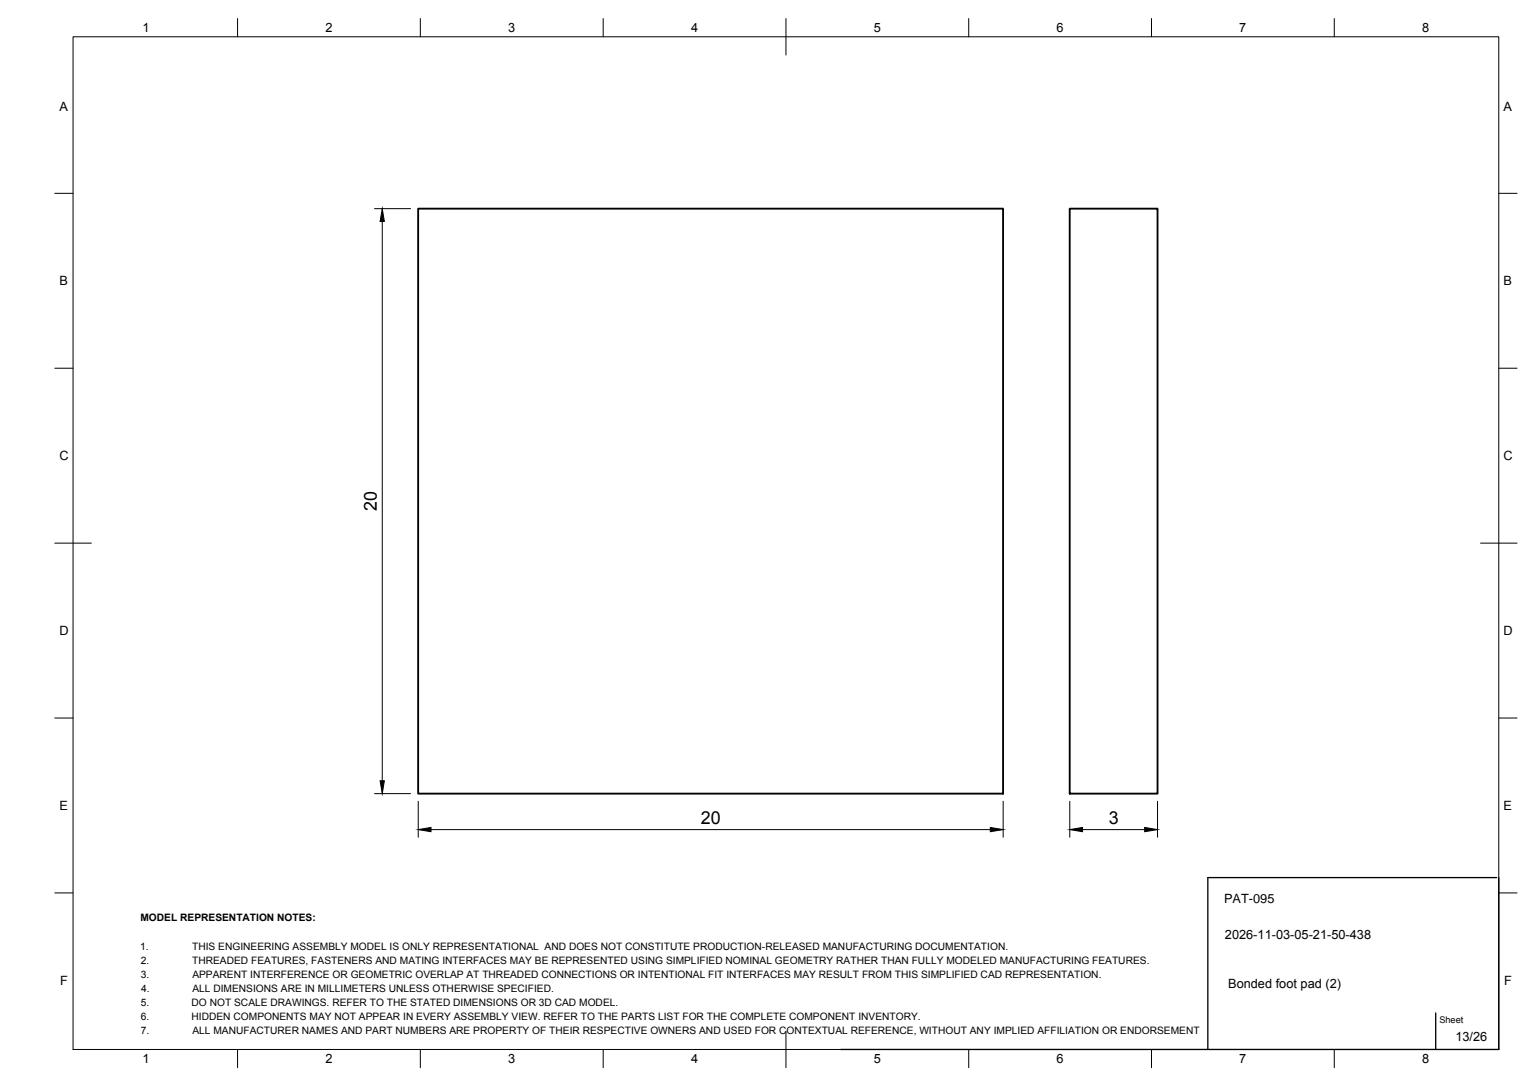
ISO-10303-21;
HEADER;
/* Generated by software containing ST-Developer
 * from STEP Tools, Inc. (www.steptools.com) 
 */

FILE_DESCRIPTION(
/* description */ ('Single-Axis Profile-Rail Linear Slide'),
/* implementation_level */ '2;1');

FILE_NAME(
/* name */ 'Bonded foot pad (2).step',
/* time_stamp */ '2026-10-27T10:47:43-07:00',
/* author */ (''),
/* organization */ (''),
/* preprocessor_version */ 'ST-DEVELOPER v20.2',
/* originating_system */ 'Autodesk Translation Framework v15.17.0.0',
/* authorisation */ '');

FILE_SCHEMA (('AUTOMOTIVE_DESIGN { 1 0 10303 214 3 1 1 }'));
ENDSEC;

DATA;
#10=MECHANICAL_DESIGN_GEOMETRIC_PRESENTATION_REPRESENTATION('',(#337),#14478);
#283=SHAPE_REPRESENTATION_RELATIONSHIP('SRR','None',#14613,#310);
#310=ADVANCED_BREP_SHAPE_REPRESENTATION('',(#364),#14457);
#337=STYLED_ITEM('',(#14824),#364);
#364=MANIFOLD_SOLID_BREP('Body1',#8597);
#636=PLANE('',#9170);
#637=PLANE('',#9171);
#638=PLANE('',#9172);
#639=PLANE('',#9173);
#640=PLANE('',#9174);
#641=PLANE('',#9175);
#1032=FACE_OUTER_BOUND('',#1531,.T.);
#1033=FACE_OUTER_BOUND('',#1532,.T.);
#1034=FACE_OUTER_BOUND('',#1533,.T.);
#1035=FACE_OUTER_BOUND('',#1534,.T.);
#1036=FACE_OUTER_BOUND('',#1535,.T.);
#1037=FACE_OUTER_BOUND('',#1536,.T.);
#1531=EDGE_LOOP('',(#6845,#6846,#6847,#6848));
#1532=EDGE_LOOP('',(#6849,#6850,#6851,#6852));
#1533=EDGE_LOOP('',(#6853,#6854,#6855,#6856));
#1534=EDGE_LOOP('',(#6857,#6858,#6859,#6860));
#1535=EDGE_LOOP('',(#6861,#6862,#6863,#6864));
#1536=EDGE_LOOP('',(#6865,#6866,#6867,#6868));
#2308=LINE('',#13062,#3279);
#2309=LINE('',#13064,#3280);
#2310=LINE('',#13066,#3281);
#2311=LINE('',#13067,#3282);
#2312=LINE('',#13070,#3283);
#2313=LINE('',#13072,#3284);
#2314=LINE('',#13073,#3285);
#2315=LINE('',#13076,#3286);
#2316=LINE('',#13078,#3287);
#2317=LINE('',#13079,#3288);
#2318=LINE('',#13081,#3289);
#2319=LINE('',#13082,#3290);
#3279=VECTOR('',#10593,1.);
#3280=VECTOR('',#10594,1.);
#3281=VECTOR('',#10595,1.);
#3282=VECTOR('',#10596,1.);
#3283=VECTOR('',#10599,1.);
#3284=VECTOR('',#10600,1.);
#3285=VECTOR('',#10601,1.);
#3286=VECTOR('',#10604,1.);
#3287=VECTOR('',#10605,1.);
#3288=VECTOR('',#10606,1.);
#3289=VECTOR('',#10609,1.);
#3290=VECTOR('',#10610,1.);
#4282=VERTEX_POINT('',#13060);
#4283=VERTEX_POINT('',#13061);
#4284=VERTEX_POINT('',#13063);
#4285=VERTEX_POINT('',#13065);
#4286=VERTEX_POINT('',#13069);
#4287=VERTEX_POINT('',#13071);
#4288=VERTEX_POINT('',#13075);
#4289=VERTEX_POINT('',#13077);
#5200=EDGE_CURVE('',#4282,#4283,#2308,.T.);
#5201=EDGE_CURVE('',#4283,#4284,#2309,.T.);
#5202=EDGE_CURVE('',#4285,#4284,#2310,.T.);
#5203=EDGE_CURVE('',#4282,#4285,#2311,.T.);
#5204=EDGE_CURVE('',#4286,#4282,#2312,.T.);
#5205=EDGE_CURVE('',#4287,#4285,#2313,.T.);
#5206=EDGE_CURVE('',#4286,#4287,#2314,.T.);
#5207=EDGE_CURVE('',#4288,#4286,#2315,.T.);
#5208=EDGE_CURVE('',#4289,#4287,#2316,.T.);
#5209=EDGE_CURVE('',#4288,#4289,#2317,.T.);
#5210=EDGE_CURVE('',#4283,#4288,#2318,.T.);
#5211=EDGE_CURVE('',#4284,#4289,#2319,.T.);
#6845=ORIENTED_EDGE('',*,*,#5200,.T.);
#6846=ORIENTED_EDGE('',*,*,#5201,.T.);
#6847=ORIENTED_EDGE('',*,*,#5202,.F.);
#6848=ORIENTED_EDGE('',*,*,#5203,.F.);
#6849=ORIENTED_EDGE('',*,*,#5204,.T.);
#6850=ORIENTED_EDGE('',*,*,#5203,.T.);
#6851=ORIENTED_EDGE('',*,*,#5205,.F.);
#6852=ORIENTED_EDGE('',*,*,#5206,.F.);
#6853=ORIENTED_EDGE('',*,*,#5207,.T.);
#6854=ORIENTED_EDGE('',*,*,#5206,.T.);
#6855=ORIENTED_EDGE('',*,*,#5208,.F.);
#6856=ORIENTED_EDGE('',*,*,#5209,.F.);
#6857=ORIENTED_EDGE('',*,*,#5210,.T.);
#6858=ORIENTED_EDGE('',*,*,#5209,.T.);
#6859=ORIENTED_EDGE('',*,*,#5211,.F.);
#6860=ORIENTED_EDGE('',*,*,#5201,.F.);
#6861=ORIENTED_EDGE('',*,*,#5211,.T.);
#6862=ORIENTED_EDGE('',*,*,#5208,.T.);
#6863=ORIENTED_EDGE('',*,*,#5205,.T.);
#6864=ORIENTED_EDGE('',*,*,#5202,.T.);
#6865=ORIENTED_EDGE('',*,*,#5210,.F.);
#6866=ORIENTED_EDGE('',*,*,#5200,.F.);
#6867=ORIENTED_EDGE('',*,*,#5204,.F.);
#6868=ORIENTED_EDGE('',*,*,#5207,.F.);
#8326=ADVANCED_FACE('',(#1032),#636,.T.);
#8327=ADVANCED_FACE('',(#1033),#637,.T.);
#8328=ADVANCED_FACE('',(#1034),#638,.T.);
#8329=ADVANCED_FACE('',(#1035),#639,.T.);
#8330=ADVANCED_FACE('',(#1036),#640,.T.);
#8331=ADVANCED_FACE('',(#1037),#641,.F.);
#8597=CLOSED_SHELL('',(#8326,#8327,#8328,#8329,#8330,#8331));
#9169=AXIS2_PLACEMENT_3D('',#13058,#10589,#10590);
#9170=AXIS2_PLACEMENT_3D('',#13059,#10591,#10592);
#9171=AXIS2_PLACEMENT_3D('',#13068,#10597,#10598);
#9172=AXIS2_PLACEMENT_3D('',#13074,#10602,#10603);
#9173=AXIS2_PLACEMENT_3D('',#13080,#10607,#10608);
#9174=AXIS2_PLACEMENT_3D('',#13083,#10611,#10612);
#9175=AXIS2_PLACEMENT_3D('',#13084,#10613,#10614);
#10589=DIRECTION('axis',(0.,0.,1.));
#10590=DIRECTION('refdir',(1.,0.,0.));
#10591=DIRECTION('center_axis',(0.,1.,0.));
#10592=DIRECTION('ref_axis',(-1.,0.,0.));
#10593=DIRECTION('',(-1.,0.,0.));
#10594=DIRECTION('',(0.,0.,1.));
#10595=DIRECTION('',(-1.,0.,0.));
#10596=DIRECTION('',(0.,0.,1.));
#10597=DIRECTION('center_axis',(1.,0.,0.));
#10598=DIRECTION('ref_axis',(0.,1.,0.));
#10599=DIRECTION('',(0.,1.,0.));
#10600=DIRECTION('',(0.,1.,0.));
#10601=DIRECTION('',(0.,0.,1.));
#10602=DIRECTION('center_axis',(0.,-1.,0.));
#10603=DIRECTION('ref_axis',(1.,0.,0.));
#10604=DIRECTION('',(1.,0.,0.));
#10605=DIRECTION('',(1.,0.,0.));
#10606=DIRECTION('',(0.,0.,1.));
#10607=DIRECTION('center_axis',(-1.,0.,0.));
#10608=DIRECTION('ref_axis',(0.,-1.,0.));
#10609=DIRECTION('',(0.,-1.,0.));
#10610=DIRECTION('',(0.,-1.,0.));
#10611=DIRECTION('center_axis',(0.,0.,1.));
#10612=DIRECTION('ref_axis',(1.,0.,0.));
#10613=DIRECTION('center_axis',(0.,0.,1.));
#10614=DIRECTION('ref_axis',(1.,0.,0.));
#13058=CARTESIAN_POINT('',(0.,0.,0.));
#13059=CARTESIAN_POINT('Origin',(20.,-2.5,-0.3));
#13060=CARTESIAN_POINT('',(20.,-2.5,-0.3));
#13061=CARTESIAN_POINT('',(18.,-2.5,-0.3));
#13062=CARTESIAN_POINT('',(20.,-2.5,-0.3));
#13063=CARTESIAN_POINT('',(18.,-2.5,0.));
#13064=CARTESIAN_POINT('',(18.,-2.5,-0.3));
#13065=CARTESIAN_POINT('',(20.,-2.5,0.));
#13066=CARTESIAN_POINT('',(20.,-2.5,0.));
#13067=CARTESIAN_POINT('',(20.,-2.5,-0.3));
#13068=CARTESIAN_POINT('Origin',(20.,-4.5,-0.3));
#13069=CARTESIAN_POINT('',(20.,-4.5,-0.3));
#13070=CARTESIAN_POINT('',(20.,-4.5,-0.3));
#13071=CARTESIAN_POINT('',(20.,-4.5,0.));
#13072=CARTESIAN_POINT('',(20.,-4.5,0.));
#13073=CARTESIAN_POINT('',(20.,-4.5,-0.3));
#13074=CARTESIAN_POINT('Origin',(18.,-4.5,-0.3));
#13075=CARTESIAN_POINT('',(18.,-4.5,-0.3));
#13076=CARTESIAN_POINT('',(18.,-4.5,-0.3));
#13077=CARTESIAN_POINT('',(18.,-4.5,0.));
#13078=CARTESIAN_POINT('',(18.,-4.5,0.));
#13079=CARTESIAN_POINT('',(18.,-4.5,-0.3));
#13080=CARTESIAN_POINT('Origin',(18.,-2.5,-0.3));
#13081=CARTESIAN_POINT('',(18.,-2.5,-0.3));
#13082=CARTESIAN_POINT('',(18.,-2.5,0.));
#13083=CARTESIAN_POINT('Origin',(19.,-3.5,0.));
#13084=CARTESIAN_POINT('Origin',(19.,-3.5,-0.3));
#14425=UNCERTAINTY_MEASURE_WITH_UNIT(LENGTH_MEASURE(0.001),#14479,
'DISTANCE_ACCURACY_VALUE',
'Maximum model space distance between geometric entities at asserted c
onnectivities');
#14446=UNCERTAINTY_MEASURE_WITH_UNIT(LENGTH_MEASURE(0.001),#14479,
'DISTANCE_ACCURACY_VALUE',
'Maximum model space distance between geometric entities at asserted c
onnectivities');
#14457=(
GEOMETRIC_REPRESENTATION_CONTEXT(3)
GLOBAL_UNCERTAINTY_ASSIGNED_CONTEXT((#14425))
GLOBAL_UNIT_ASSIGNED_CONTEXT((#14479,#14481,#14482))
REPRESENTATION_CONTEXT('','3D')
);
#14478=(
GEOMETRIC_REPRESENTATION_CONTEXT(3)
GLOBAL_UNCERTAINTY_ASSIGNED_CONTEXT((#14446))
GLOBAL_UNIT_ASSIGNED_CONTEXT((#14479,#14481,#14482))
REPRESENTATION_CONTEXT('','3D')
);
#14479=(
LENGTH_UNIT()
NAMED_UNIT(*)
SI_UNIT(.CENTI.,.METRE.)
);
#14481=(
NAMED_UNIT(*)
PLANE_ANGLE_UNIT()
SI_UNIT($,.RADIAN.)
);
#14482=(
NAMED_UNIT(*)
SI_UNIT($,.STERADIAN.)
SOLID_ANGLE_UNIT()
);
#14493=SHAPE_DEFINITION_REPRESENTATION(#14524,#14613);
#14524=PRODUCT_DEFINITION_SHAPE('',$,#14645);
#14613=SHAPE_REPRESENTATION('',(#9169),#14457);
#14634=PRODUCT_DEFINITION_CONTEXT('part definition',#14729,'design');
#14645=PRODUCT_DEFINITION('Bonded foot pad (2)','Bonded foot pad (2)',#14676,
#14634);
#14676=PRODUCT_DEFINITION_FORMATION('',$,#14741);
#14729=APPLICATION_CONTEXT(
'Core Data for Automotive Mechanical Design Process');
#14730=PRODUCT_CONTEXT('part definition',#14729,'mechanical');
#14741=PRODUCT('Bonded foot pad (2)','Bonded foot pad (2)',
'Bonded foot pad (2)',(#14730));
#14818=COLOUR_RGB('Sky Blue',0.24,0.69,0.87);
#14819=FILL_AREA_STYLE_COLOUR('',#14818);
#14820=FILL_AREA_STYLE('',(#14819));
#14821=SURFACE_STYLE_FILL_AREA(#14820);
#14822=SURFACE_SIDE_STYLE('',(#14821));
#14823=SURFACE_STYLE_USAGE(.BOTH.,#14822);
#14824=PRESENTATION_STYLE_ASSIGNMENT((#14823));
ENDSEC;
END-ISO-10303-21;
